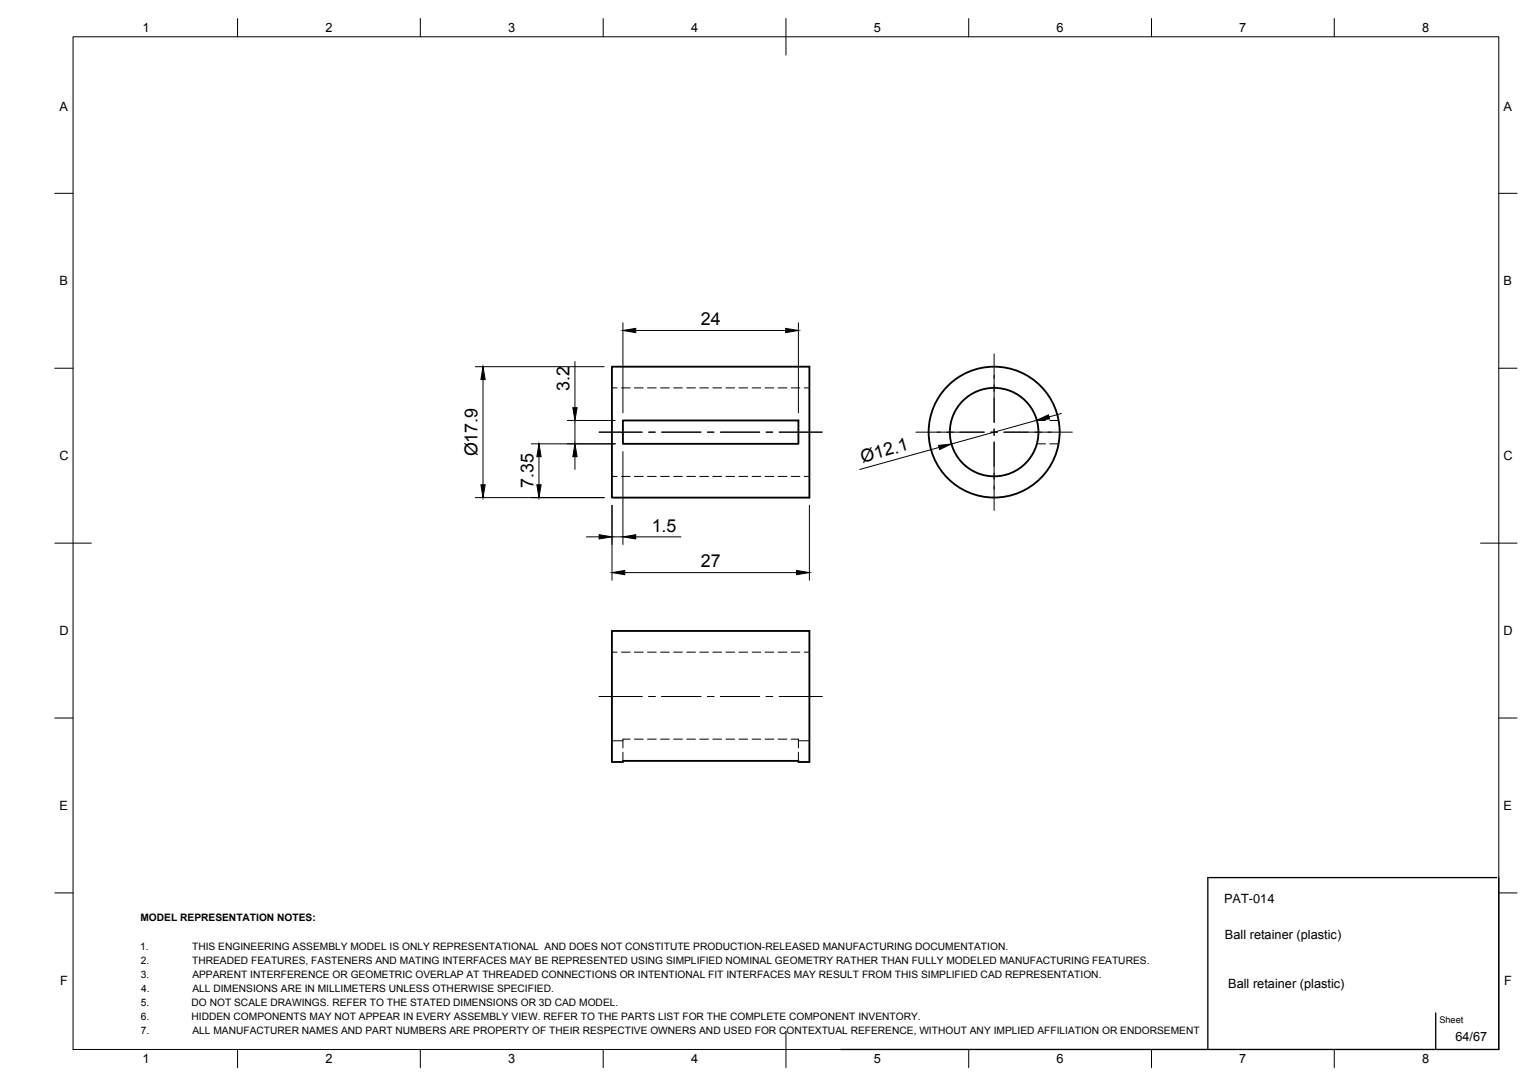
ISO-10303-21;
HEADER;
/* Generated by software containing ST-Developer
 * from STEP Tools, Inc. (www.steptools.com) 
 */

FILE_DESCRIPTION(
/* description */ ('Bin tilter linkage'),
/* implementation_level */ '2;1');

FILE_NAME(
/* name */ 'Ball retainer (plastic).step',
/* time_stamp */ '2026-10-28T03:26:24-07:00',
/* author */ (''),
/* organization */ (''),
/* preprocessor_version */ 'ST-DEVELOPER v20.2',
/* originating_system */ 'Autodesk Translation Framework v15.17.0.0',
/* authorisation */ '');

FILE_SCHEMA (('AUTOMOTIVE_DESIGN { 1 0 10303 214 3 1 1 }'));
ENDSEC;

DATA;
#10=MECHANICAL_DESIGN_GEOMETRIC_PRESENTATION_REPRESENTATION('',(#968),#23728);
#748=SHAPE_REPRESENTATION_RELATIONSHIP('SRR','None',#24218,#854);
#854=ADVANCED_BREP_SHAPE_REPRESENTATION('',(#1080),#23718);
#968=STYLED_ITEM('',(#24758),#1080);
#1080=MANIFOLD_SOLID_BREP('Body1',#12500);
#1477=FACE_BOUND('',#3789,.T.);
#1478=FACE_BOUND('',#3791,.T.);
#1479=FACE_BOUND('',#3793,.T.);
#1480=FACE_BOUND('',#3795,.T.);
#1859=PLANE('',#15351);
#1860=PLANE('',#15354);
#1861=PLANE('',#15355);
#1862=PLANE('',#15358);
#1863=PLANE('',#15359);
#1864=PLANE('',#15364);
#2617=FACE_OUTER_BOUND('',#3784,.T.);
#2618=FACE_OUTER_BOUND('',#3785,.T.);
#2619=FACE_OUTER_BOUND('',#3786,.T.);
#2620=FACE_OUTER_BOUND('',#3787,.T.);
#2621=FACE_OUTER_BOUND('',#3788,.T.);
#2622=FACE_OUTER_BOUND('',#3790,.T.);
#2623=FACE_OUTER_BOUND('',#3792,.T.);
#2624=FACE_OUTER_BOUND('',#3794,.T.);
#3784=EDGE_LOOP('',(#11087,#11088,#11089,#11090));
#3785=EDGE_LOOP('',(#11091,#11092,#11093,#11094));
#3786=EDGE_LOOP('',(#11095,#11096,#11097,#11098));
#3787=EDGE_LOOP('',(#11099,#11100,#11101,#11102));
#3788=EDGE_LOOP('',(#11103));
#3789=EDGE_LOOP('',(#11104));
#3790=EDGE_LOOP('',(#11105,#11106,#11107,#11108));
#3791=EDGE_LOOP('',(#11109,#11110,#11111,#11112));
#3792=EDGE_LOOP('',(#11113));
#3793=EDGE_LOOP('',(#11114));
#3794=EDGE_LOOP('',(#11115,#11116,#11117,#11118));
#3795=EDGE_LOOP('',(#11119,#11120,#11121,#11122));
#4473=LINE('',#23267,#5148);
#4474=LINE('',#23270,#5149);
#4475=LINE('',#23273,#5150);
#4476=LINE('',#23275,#5151);
#4477=LINE('',#23276,#5152);
#4478=LINE('',#23282,#5153);
#4479=LINE('',#23284,#5154);
#4480=LINE('',#23285,#5155);
#4481=LINE('',#23294,#5156);
#4482=LINE('',#23299,#5157);
#5148=VECTOR('',#19452,1.);
#5149=VECTOR('',#19455,1.);
#5150=VECTOR('',#19458,1.);
#5151=VECTOR('',#19459,1.);
#5152=VECTOR('',#19460,1.);
#5153=VECTOR('',#19467,1.);
#5154=VECTOR('',#19470,1.);
#5155=VECTOR('',#19471,1.);
#5156=VECTOR('',#19482,0.895);
#5157=VECTOR('',#19489,0.605);
#5918=CIRCLE('',#15352,0.895);
#5919=CIRCLE('',#15353,0.605);
#5920=CIRCLE('',#15356,0.895);
#5921=CIRCLE('',#15357,0.605);
#5922=CIRCLE('',#15360,0.895);
#5923=CIRCLE('',#15361,0.605);
#5924=CIRCLE('',#15363,0.895);
#5925=CIRCLE('',#15365,0.605);
#6867=VERTEX_POINT('',#23263);
#6868=VERTEX_POINT('',#23264);
#6869=VERTEX_POINT('',#23266);
#6870=VERTEX_POINT('',#23268);
#6871=VERTEX_POINT('',#23272);
#6872=VERTEX_POINT('',#23274);
#6873=VERTEX_POINT('',#23278);
#6874=VERTEX_POINT('',#23280);
#6875=VERTEX_POINT('',#23287);
#6876=VERTEX_POINT('',#23289);
#6877=VERTEX_POINT('',#23292);
#6878=VERTEX_POINT('',#23296);
#8283=EDGE_CURVE('',#6867,#6868,#5918,.T.);
#8284=EDGE_CURVE('',#6869,#6867,#4473,.T.);
#8285=EDGE_CURVE('',#6870,#6869,#5919,.T.);
#8286=EDGE_CURVE('',#6868,#6870,#4474,.T.);
#8287=EDGE_CURVE('',#6868,#6871,#4475,.T.);
#8288=EDGE_CURVE('',#6872,#6870,#4476,.T.);
#8289=EDGE_CURVE('',#6872,#6871,#4477,.T.);
#8290=EDGE_CURVE('',#6871,#6873,#5920,.T.);
#8291=EDGE_CURVE('',#6874,#6872,#5921,.T.);
#8292=EDGE_CURVE('',#6873,#6874,#4478,.T.);
#8293=EDGE_CURVE('',#6873,#6867,#4479,.T.);
#8294=EDGE_CURVE('',#6869,#6874,#4480,.T.);
#8295=EDGE_CURVE('',#6875,#6875,#5922,.T.);
#8296=EDGE_CURVE('',#6876,#6876,#5923,.T.);
#8297=EDGE_CURVE('',#6877,#6877,#5924,.T.);
#8298=EDGE_CURVE('',#6877,#6875,#4481,.T.);
#8299=EDGE_CURVE('',#6878,#6878,#5925,.T.);
#8300=EDGE_CURVE('',#6878,#6876,#4482,.T.);
#11087=ORIENTED_EDGE('',*,*,#8283,.F.);
#11088=ORIENTED_EDGE('',*,*,#8284,.F.);
#11089=ORIENTED_EDGE('',*,*,#8285,.F.);
#11090=ORIENTED_EDGE('',*,*,#8286,.F.);
#11091=ORIENTED_EDGE('',*,*,#8287,.F.);
#11092=ORIENTED_EDGE('',*,*,#8286,.T.);
#11093=ORIENTED_EDGE('',*,*,#8288,.F.);
#11094=ORIENTED_EDGE('',*,*,#8289,.T.);
#11095=ORIENTED_EDGE('',*,*,#8290,.F.);
#11096=ORIENTED_EDGE('',*,*,#8289,.F.);
#11097=ORIENTED_EDGE('',*,*,#8291,.F.);
#11098=ORIENTED_EDGE('',*,*,#8292,.F.);
#11099=ORIENTED_EDGE('',*,*,#8293,.F.);
#11100=ORIENTED_EDGE('',*,*,#8292,.T.);
#11101=ORIENTED_EDGE('',*,*,#8294,.F.);
#11102=ORIENTED_EDGE('',*,*,#8284,.T.);
#11103=ORIENTED_EDGE('',*,*,#8295,.F.);
#11104=ORIENTED_EDGE('',*,*,#8296,.T.);
#11105=ORIENTED_EDGE('',*,*,#8297,.F.);
#11106=ORIENTED_EDGE('',*,*,#8298,.T.);
#11107=ORIENTED_EDGE('',*,*,#8295,.T.);
#11108=ORIENTED_EDGE('',*,*,#8298,.F.);
#11109=ORIENTED_EDGE('',*,*,#8290,.T.);
#11110=ORIENTED_EDGE('',*,*,#8293,.T.);
#11111=ORIENTED_EDGE('',*,*,#8283,.T.);
#11112=ORIENTED_EDGE('',*,*,#8287,.T.);
#11113=ORIENTED_EDGE('',*,*,#8297,.T.);
#11114=ORIENTED_EDGE('',*,*,#8299,.F.);
#11115=ORIENTED_EDGE('',*,*,#8299,.T.);
#11116=ORIENTED_EDGE('',*,*,#8300,.T.);
#11117=ORIENTED_EDGE('',*,*,#8296,.F.);
#11118=ORIENTED_EDGE('',*,*,#8300,.F.);
#11119=ORIENTED_EDGE('',*,*,#8291,.T.);
#11120=ORIENTED_EDGE('',*,*,#8288,.T.);
#11121=ORIENTED_EDGE('',*,*,#8285,.T.);
#11122=ORIENTED_EDGE('',*,*,#8294,.T.);
#11599=CYLINDRICAL_SURFACE('',#15362,0.895);
#11600=CYLINDRICAL_SURFACE('',#15366,0.605);
#12342=ADVANCED_FACE('',(#2617),#1859,.F.);
#12343=ADVANCED_FACE('',(#2618),#1860,.F.);
#12344=ADVANCED_FACE('',(#2619),#1861,.F.);
#12345=ADVANCED_FACE('',(#2620),#1862,.F.);
#12346=ADVANCED_FACE('',(#2621,#1477),#1863,.T.);
#12347=ADVANCED_FACE('',(#2622,#1478),#11599,.T.);
#12348=ADVANCED_FACE('',(#2623,#1479),#1864,.T.);
#12349=ADVANCED_FACE('',(#2624,#1480),#11600,.F.);
#12500=CLOSED_SHELL('',(#12342,#12343,#12344,#12345,#12346,#12347,#12348,
#12349));
#15350=AXIS2_PLACEMENT_3D('',#23261,#19446,#19447);
#15351=AXIS2_PLACEMENT_3D('',#23262,#19448,#19449);
#15352=AXIS2_PLACEMENT_3D('',#23265,#19450,#19451);
#15353=AXIS2_PLACEMENT_3D('',#23269,#19453,#19454);
#15354=AXIS2_PLACEMENT_3D('',#23271,#19456,#19457);
#15355=AXIS2_PLACEMENT_3D('',#23277,#19461,#19462);
#15356=AXIS2_PLACEMENT_3D('',#23279,#19463,#19464);
#15357=AXIS2_PLACEMENT_3D('',#23281,#19465,#19466);
#15358=AXIS2_PLACEMENT_3D('',#23283,#19468,#19469);
#15359=AXIS2_PLACEMENT_3D('',#23286,#19472,#19473);
#15360=AXIS2_PLACEMENT_3D('',#23288,#19474,#19475);
#15361=AXIS2_PLACEMENT_3D('',#23290,#19476,#19477);
#15362=AXIS2_PLACEMENT_3D('',#23291,#19478,#19479);
#15363=AXIS2_PLACEMENT_3D('',#23293,#19480,#19481);
#15364=AXIS2_PLACEMENT_3D('',#23295,#19483,#19484);
#15365=AXIS2_PLACEMENT_3D('',#23297,#19485,#19486);
#15366=AXIS2_PLACEMENT_3D('',#23298,#19487,#19488);
#19446=DIRECTION('axis',(0.,0.,1.));
#19447=DIRECTION('refdir',(1.,0.,0.));
#19448=DIRECTION('center_axis',(0.,1.,0.));
#19449=DIRECTION('ref_axis',(0.,0.,1.));
#19450=DIRECTION('center_axis',(0.,1.,0.));
#19451=DIRECTION('ref_axis',(1.,0.,0.));
#19452=DIRECTION('',(1.,0.,0.));
#19453=DIRECTION('center_axis',(0.,-1.,0.));
#19454=DIRECTION('ref_axis',(1.,0.,0.));
#19455=DIRECTION('',(-1.,0.,0.));
#19456=DIRECTION('center_axis',(0.,0.,-1.));
#19457=DIRECTION('ref_axis',(-1.,0.,0.));
#19458=DIRECTION('',(0.,-1.,0.));
#19459=DIRECTION('',(0.,1.,0.));
#19460=DIRECTION('',(1.,0.,0.));
#19461=DIRECTION('center_axis',(0.,-1.,0.));
#19462=DIRECTION('ref_axis',(0.,0.,-1.));
#19463=DIRECTION('center_axis',(0.,-1.,0.));
#19464=DIRECTION('ref_axis',(1.,0.,0.));
#19465=DIRECTION('center_axis',(0.,1.,0.));
#19466=DIRECTION('ref_axis',(1.,0.,0.));
#19467=DIRECTION('',(-1.,0.,0.));
#19468=DIRECTION('center_axis',(0.,0.,1.));
#19469=DIRECTION('ref_axis',(1.,0.,0.));
#19470=DIRECTION('',(0.,1.,0.));
#19471=DIRECTION('',(0.,-1.,0.));
#19472=DIRECTION('center_axis',(0.,1.,0.));
#19473=DIRECTION('ref_axis',(0.,0.,1.));
#19474=DIRECTION('center_axis',(0.,-1.,0.));
#19475=DIRECTION('ref_axis',(1.,0.,0.));
#19476=DIRECTION('center_axis',(0.,-1.,0.));
#19477=DIRECTION('ref_axis',(1.,0.,0.));
#19478=DIRECTION('center_axis',(0.,-1.,0.));
#19479=DIRECTION('ref_axis',(1.,0.,0.));
#19480=DIRECTION('center_axis',(0.,-1.,0.));
#19481=DIRECTION('ref_axis',(1.,0.,0.));
#19482=DIRECTION('',(0.,1.,0.));
#19483=DIRECTION('center_axis',(0.,-1.,0.));
#19484=DIRECTION('ref_axis',(0.,0.,-1.));
#19485=DIRECTION('center_axis',(0.,-1.,0.));
#19486=DIRECTION('ref_axis',(1.,0.,0.));
#19487=DIRECTION('center_axis',(0.,-1.,0.));
#19488=DIRECTION('ref_axis',(1.,0.,0.));
#19489=DIRECTION('',(0.,1.,0.));
#23261=CARTESIAN_POINT('',(0.,0.,0.));
#23262=CARTESIAN_POINT('Origin',(0.75,1.2,0.));
#23263=CARTESIAN_POINT('',(0.880582193778639,1.2,0.16));
#23264=CARTESIAN_POINT('',(0.880582193778639,1.2,-0.16));
#23265=CARTESIAN_POINT('Origin',(0.,1.2,0.));
#23266=CARTESIAN_POINT('',(0.583459510163302,1.2,0.16));
#23267=CARTESIAN_POINT('',(0.57,1.2,0.16));
#23268=CARTESIAN_POINT('',(0.583459510163302,1.2,-0.16));
#23269=CARTESIAN_POINT('Origin',(0.,1.2,0.));
#23270=CARTESIAN_POINT('',(0.93,1.2,-0.16));
#23271=CARTESIAN_POINT('Origin',(0.93,0.,-0.16));
#23272=CARTESIAN_POINT('',(0.880582193778639,-1.2,-0.16));
#23273=CARTESIAN_POINT('',(0.880582193778639,0.,-0.16));
#23274=CARTESIAN_POINT('',(0.583459510163302,-1.2,-0.16));
#23275=CARTESIAN_POINT('',(0.583459510163302,0.,-0.16));
#23276=CARTESIAN_POINT('',(0.93,-1.2,-0.16));
#23277=CARTESIAN_POINT('Origin',(0.75,-1.2,0.));
#23278=CARTESIAN_POINT('',(0.880582193778639,-1.2,0.16));
#23279=CARTESIAN_POINT('Origin',(0.,-1.2,0.));
#23280=CARTESIAN_POINT('',(0.583459510163302,-1.2,0.16));
#23281=CARTESIAN_POINT('Origin',(0.,-1.2,0.));
#23282=CARTESIAN_POINT('',(0.57,-1.2,0.16));
#23283=CARTESIAN_POINT('Origin',(0.57,0.,0.16));
#23284=CARTESIAN_POINT('',(0.880582193778639,0.,0.16));
#23285=CARTESIAN_POINT('',(0.583459510163302,0.,0.16));
#23286=CARTESIAN_POINT('Origin',(0.895,1.35,0.));
#23287=CARTESIAN_POINT('',(-0.895,1.35,-1.09605888523688E-16));
#23288=CARTESIAN_POINT('Origin',(0.,1.35,0.));
#23289=CARTESIAN_POINT('',(-0.605,1.35,-7.40911313484149E-17));
#23290=CARTESIAN_POINT('Origin',(0.,1.35,0.));
#23291=CARTESIAN_POINT('Origin',(0.,0.,0.));
#23292=CARTESIAN_POINT('',(-0.895,-1.35,-1.09605888523688E-16));
#23293=CARTESIAN_POINT('Origin',(0.,-1.35,0.));
#23294=CARTESIAN_POINT('',(-0.895,0.,-1.09605888523688E-16));
#23295=CARTESIAN_POINT('Origin',(0.605,-1.35,0.));
#23296=CARTESIAN_POINT('',(-0.605,-1.35,-7.40911313484149E-17));
#23297=CARTESIAN_POINT('Origin',(0.,-1.35,0.));
#23298=CARTESIAN_POINT('Origin',(0.,0.,0.));
#23299=CARTESIAN_POINT('',(-0.605,0.,-7.40911313484149E-17));
#23601=UNCERTAINTY_MEASURE_WITH_UNIT(LENGTH_MEASURE(0.001),#23729,
'DISTANCE_ACCURACY_VALUE',
'Maximum model space distance between geometric entities at asserted c
onnectivities');
#23611=UNCERTAINTY_MEASURE_WITH_UNIT(LENGTH_MEASURE(0.001),#23729,
'DISTANCE_ACCURACY_VALUE',
'Maximum model space distance between geometric entities at asserted c
onnectivities');
#23718=(
GEOMETRIC_REPRESENTATION_CONTEXT(3)
GLOBAL_UNCERTAINTY_ASSIGNED_CONTEXT((#23601))
GLOBAL_UNIT_ASSIGNED_CONTEXT((#23729,#23731,#23732))
REPRESENTATION_CONTEXT('','3D')
);
#23728=(
GEOMETRIC_REPRESENTATION_CONTEXT(3)
GLOBAL_UNCERTAINTY_ASSIGNED_CONTEXT((#23611))
GLOBAL_UNIT_ASSIGNED_CONTEXT((#23729,#23731,#23732))
REPRESENTATION_CONTEXT('','3D')
);
#23729=(
LENGTH_UNIT()
NAMED_UNIT(*)
SI_UNIT(.CENTI.,.METRE.)
);
#23731=(
NAMED_UNIT(*)
PLANE_ANGLE_UNIT()
SI_UNIT($,.RADIAN.)
);
#23732=(
NAMED_UNIT(*)
SI_UNIT($,.STERADIAN.)
SOLID_ANGLE_UNIT()
);
#23839=SHAPE_DEFINITION_REPRESENTATION(#24077,#24218);
#24077=PRODUCT_DEFINITION_SHAPE('',$,#24335);
#24218=SHAPE_REPRESENTATION('',(#15350),#23718);
#24228=PRODUCT_DEFINITION_CONTEXT('part definition',#24578,'design');
#24335=PRODUCT_DEFINITION('Ball retainer (plastic)',
'Ball retainer (plastic)',#24451,#24228);
#24451=PRODUCT_DEFINITION_FORMATION('',$,#24686);
#24578=APPLICATION_CONTEXT(
'Core Data for Automotive Mechanical Design Process');
#24579=PRODUCT_CONTEXT('part definition',#24578,'mechanical');
#24686=PRODUCT('Ball retainer (plastic)','Ball retainer (plastic)',
'Ball retainer (plastic)',(#24579));
#24752=COLOUR_RGB('Sky Blue',0.24,0.69,0.87);
#24753=FILL_AREA_STYLE_COLOUR('',#24752);
#24754=FILL_AREA_STYLE('',(#24753));
#24755=SURFACE_STYLE_FILL_AREA(#24754);
#24756=SURFACE_SIDE_STYLE('',(#24755));
#24757=SURFACE_STYLE_USAGE(.BOTH.,#24756);
#24758=PRESENTATION_STYLE_ASSIGNMENT((#24757));
ENDSEC;
END-ISO-10303-21;
